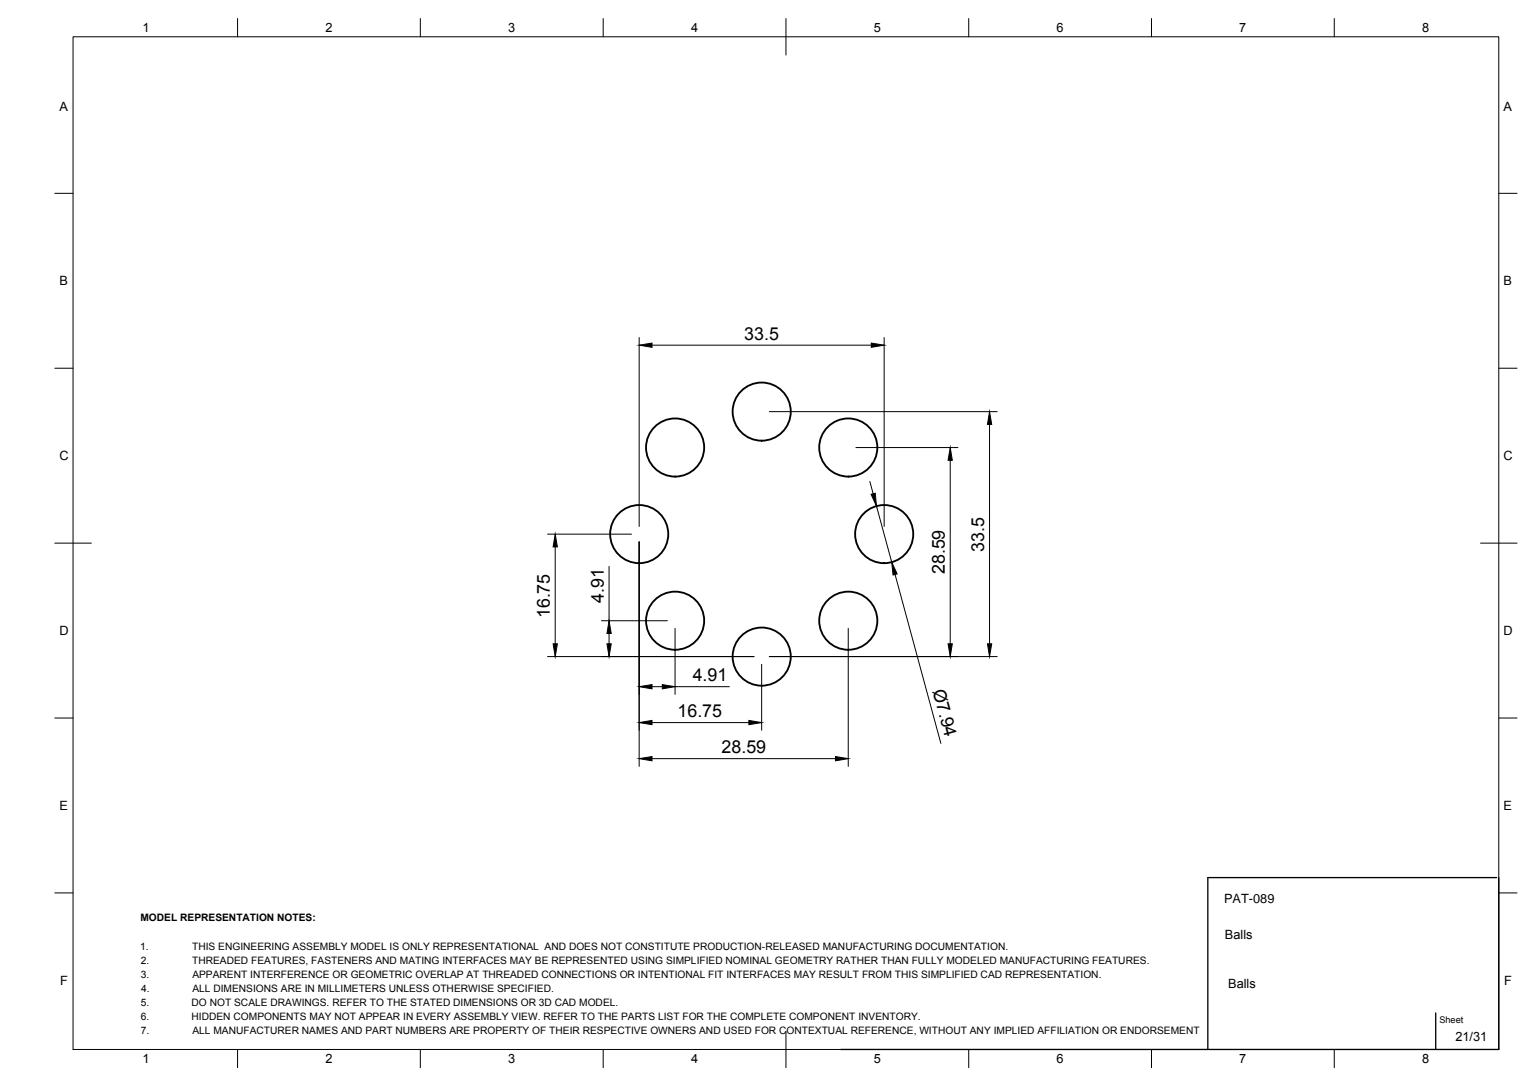
ISO-10303-21;
HEADER;
/* Generated by software containing ST-Developer
 * from STEP Tools, Inc. (www.steptools.com) 
 */

FILE_DESCRIPTION(
/* description */ ('Rotary union on bearing shaft'),
/* implementation_level */ '2;1');

FILE_NAME(
/* name */ 'Balls.step',
/* time_stamp */ '2026-10-28T03:24:01-07:00',
/* author */ (''),
/* organization */ (''),
/* preprocessor_version */ 'ST-DEVELOPER v20.2',
/* originating_system */ 'Autodesk Translation Framework v15.17.0.0',
/* authorisation */ '');

FILE_SCHEMA (('AUTOMOTIVE_DESIGN { 1 0 10303 214 3 1 1 }'));
ENDSEC;

DATA;
#10=MECHANICAL_DESIGN_GEOMETRIC_PRESENTATION_REPRESENTATION('',(#326,#327,#328,#329,#330,#331,#332,#333),#9448);
#185=SPHERICAL_SURFACE('',#5469,0.3969);
#186=SPHERICAL_SURFACE('',#5471,0.3969);
#187=SPHERICAL_SURFACE('',#5473,0.3969);
#188=SPHERICAL_SURFACE('',#5475,0.3969);
#189=SPHERICAL_SURFACE('',#5477,0.3969);
#190=SPHERICAL_SURFACE('',#5479,0.3969);
#191=SPHERICAL_SURFACE('',#5481,0.3969);
#192=SPHERICAL_SURFACE('',#5483,0.3969);
#272=SHAPE_REPRESENTATION_RELATIONSHIP('SRR','None',#9573,#299);
#299=ADVANCED_BREP_SHAPE_REPRESENTATION('',(#361,#362,#363,#364,#365,#366,
#367,#368),#9433);
#326=STYLED_ITEM('',(#9778),#361);
#327=STYLED_ITEM('',(#9778),#362);
#328=STYLED_ITEM('',(#9778),#363);
#329=STYLED_ITEM('',(#9778),#364);
#330=STYLED_ITEM('',(#9778),#365);
#331=STYLED_ITEM('',(#9778),#366);
#332=STYLED_ITEM('',(#9778),#367);
#333=STYLED_ITEM('',(#9778),#368);
#361=MANIFOLD_SOLID_BREP('Body1',#4881);
#362=MANIFOLD_SOLID_BREP('Body2',#4882);
#363=MANIFOLD_SOLID_BREP('Body3',#4883);
#364=MANIFOLD_SOLID_BREP('Body4',#4884);
#365=MANIFOLD_SOLID_BREP('Body5',#4885);
#366=MANIFOLD_SOLID_BREP('Body6',#4886);
#367=MANIFOLD_SOLID_BREP('Body7',#4887);
#368=MANIFOLD_SOLID_BREP('Body8',#4888);
#783=FACE_OUTER_BOUND('',#1150,.T.);
#784=FACE_OUTER_BOUND('',#1151,.T.);
#785=FACE_OUTER_BOUND('',#1152,.T.);
#786=FACE_OUTER_BOUND('',#1153,.T.);
#787=FACE_OUTER_BOUND('',#1154,.T.);
#788=FACE_OUTER_BOUND('',#1155,.T.);
#789=FACE_OUTER_BOUND('',#1156,.T.);
#790=FACE_OUTER_BOUND('',#1157,.T.);
#1150=EDGE_LOOP('',(#3787,#3788));
#1151=EDGE_LOOP('',(#3789,#3790));
#1152=EDGE_LOOP('',(#3791,#3792));
#1153=EDGE_LOOP('',(#3793,#3794));
#1154=EDGE_LOOP('',(#3795,#3796));
#1155=EDGE_LOOP('',(#3797,#3798));
#1156=EDGE_LOOP('',(#3799,#3800));
#1157=EDGE_LOOP('',(#3801,#3802));
#2122=CIRCLE('',#5470,0.3969);
#2123=CIRCLE('',#5472,0.3969);
#2124=CIRCLE('',#5474,0.3969);
#2125=CIRCLE('',#5476,0.3969);
#2126=CIRCLE('',#5478,0.3969);
#2127=CIRCLE('',#5480,0.3969);
#2128=CIRCLE('',#5482,0.3969);
#2129=CIRCLE('',#5484,0.3969);
#2424=VERTEX_POINT('',#8101);
#2425=VERTEX_POINT('',#8102);
#2426=VERTEX_POINT('',#8105);
#2427=VERTEX_POINT('',#8106);
#2428=VERTEX_POINT('',#8109);
#2429=VERTEX_POINT('',#8110);
#2430=VERTEX_POINT('',#8113);
#2431=VERTEX_POINT('',#8114);
#2432=VERTEX_POINT('',#8117);
#2433=VERTEX_POINT('',#8118);
#2434=VERTEX_POINT('',#8121);
#2435=VERTEX_POINT('',#8122);
#2436=VERTEX_POINT('',#8125);
#2437=VERTEX_POINT('',#8126);
#2438=VERTEX_POINT('',#8129);
#2439=VERTEX_POINT('',#8130);
#2921=EDGE_CURVE('',#2424,#2425,#2122,.T.);
#2922=EDGE_CURVE('',#2426,#2427,#2123,.T.);
#2923=EDGE_CURVE('',#2428,#2429,#2124,.T.);
#2924=EDGE_CURVE('',#2430,#2431,#2125,.T.);
#2925=EDGE_CURVE('',#2432,#2433,#2126,.T.);
#2926=EDGE_CURVE('',#2434,#2435,#2127,.T.);
#2927=EDGE_CURVE('',#2436,#2437,#2128,.T.);
#2928=EDGE_CURVE('',#2438,#2439,#2129,.T.);
#3787=ORIENTED_EDGE('',*,*,#2921,.T.);
#3788=ORIENTED_EDGE('',*,*,#2921,.F.);
#3789=ORIENTED_EDGE('',*,*,#2922,.T.);
#3790=ORIENTED_EDGE('',*,*,#2922,.F.);
#3791=ORIENTED_EDGE('',*,*,#2923,.T.);
#3792=ORIENTED_EDGE('',*,*,#2923,.F.);
#3793=ORIENTED_EDGE('',*,*,#2924,.T.);
#3794=ORIENTED_EDGE('',*,*,#2924,.F.);
#3795=ORIENTED_EDGE('',*,*,#2925,.T.);
#3796=ORIENTED_EDGE('',*,*,#2925,.F.);
#3797=ORIENTED_EDGE('',*,*,#2926,.T.);
#3798=ORIENTED_EDGE('',*,*,#2926,.F.);
#3799=ORIENTED_EDGE('',*,*,#2927,.T.);
#3800=ORIENTED_EDGE('',*,*,#2927,.F.);
#3801=ORIENTED_EDGE('',*,*,#2928,.T.);
#3802=ORIENTED_EDGE('',*,*,#2928,.F.);
#4696=ADVANCED_FACE('',(#783),#185,.T.);
#4697=ADVANCED_FACE('',(#784),#186,.T.);
#4698=ADVANCED_FACE('',(#785),#187,.T.);
#4699=ADVANCED_FACE('',(#786),#188,.T.);
#4700=ADVANCED_FACE('',(#787),#189,.T.);
#4701=ADVANCED_FACE('',(#788),#190,.T.);
#4702=ADVANCED_FACE('',(#789),#191,.T.);
#4703=ADVANCED_FACE('',(#790),#192,.T.);
#4881=CLOSED_SHELL('',(#4696));
#4882=CLOSED_SHELL('',(#4697));
#4883=CLOSED_SHELL('',(#4698));
#4884=CLOSED_SHELL('',(#4699));
#4885=CLOSED_SHELL('',(#4700));
#4886=CLOSED_SHELL('',(#4701));
#4887=CLOSED_SHELL('',(#4702));
#4888=CLOSED_SHELL('',(#4703));
#5468=AXIS2_PLACEMENT_3D('',#8099,#6487,#6488);
#5469=AXIS2_PLACEMENT_3D('',#8100,#6489,#6490);
#5470=AXIS2_PLACEMENT_3D('',#8103,#6491,#6492);
#5471=AXIS2_PLACEMENT_3D('',#8104,#6493,#6494);
#5472=AXIS2_PLACEMENT_3D('',#8107,#6495,#6496);
#5473=AXIS2_PLACEMENT_3D('',#8108,#6497,#6498);
#5474=AXIS2_PLACEMENT_3D('',#8111,#6499,#6500);
#5475=AXIS2_PLACEMENT_3D('',#8112,#6501,#6502);
#5476=AXIS2_PLACEMENT_3D('',#8115,#6503,#6504);
#5477=AXIS2_PLACEMENT_3D('',#8116,#6505,#6506);
#5478=AXIS2_PLACEMENT_3D('',#8119,#6507,#6508);
#5479=AXIS2_PLACEMENT_3D('',#8120,#6509,#6510);
#5480=AXIS2_PLACEMENT_3D('',#8123,#6511,#6512);
#5481=AXIS2_PLACEMENT_3D('',#8124,#6513,#6514);
#5482=AXIS2_PLACEMENT_3D('',#8127,#6515,#6516);
#5483=AXIS2_PLACEMENT_3D('',#8128,#6517,#6518);
#5484=AXIS2_PLACEMENT_3D('',#8131,#6519,#6520);
#6487=DIRECTION('axis',(0.,0.,1.));
#6488=DIRECTION('refdir',(1.,0.,0.));
#6489=DIRECTION('center_axis',(0.,0.,1.));
#6490=DIRECTION('ref_axis',(1.,0.,0.));
#6491=DIRECTION('center_axis',(1.22464679914735E-16,-1.,0.));
#6492=DIRECTION('ref_axis',(-1.,-1.22464679914735E-16,0.));
#6493=DIRECTION('center_axis',(0.707106781186548,0.,0.707106781186548));
#6494=DIRECTION('ref_axis',(0.707106781186548,0.,-0.707106781186548));
#6495=DIRECTION('center_axis',(8.65956056235493E-17,-1.,-8.65956056235493E-17));
#6496=DIRECTION('ref_axis',(-0.707106781186548,-1.22464679914735E-16,0.707106781186548));
#6497=DIRECTION('center_axis',(1.,0.,0.));
#6498=DIRECTION('ref_axis',(6.12323399573677E-17,0.,-1.));
#6499=DIRECTION('center_axis',(7.49879891330929E-33,-1.,-1.22464679914735E-16));
#6500=DIRECTION('ref_axis',(-6.12323399573677E-17,-1.22464679914735E-16,
1.));
#6501=DIRECTION('center_axis',(0.707106781186548,0.,-0.707106781186548));
#6502=DIRECTION('ref_axis',(-0.707106781186548,0.,-0.707106781186548));
#6503=DIRECTION('center_axis',(-8.65956056235493E-17,-1.,-8.65956056235493E-17));
#6504=DIRECTION('ref_axis',(0.707106781186548,-1.22464679914735E-16,0.707106781186548));
#6505=DIRECTION('center_axis',(0.,0.,-1.));
#6506=DIRECTION('ref_axis',(-1.,0.,-1.22464679914735E-16));
#6507=DIRECTION('center_axis',(-1.22464679914735E-16,-1.,-1.49975978266186E-32));
#6508=DIRECTION('ref_axis',(1.,-1.22464679914735E-16,1.22464679914735E-16));
#6509=DIRECTION('center_axis',(-0.707106781186548,0.,-0.707106781186548));
#6510=DIRECTION('ref_axis',(-0.707106781186548,0.,0.707106781186548));
#6511=DIRECTION('center_axis',(-8.65956056235493E-17,-1.,8.65956056235493E-17));
#6512=DIRECTION('ref_axis',(0.707106781186548,-1.22464679914735E-16,-0.707106781186548));
#6513=DIRECTION('center_axis',(-1.,0.,0.));
#6514=DIRECTION('ref_axis',(-1.83697019872103E-16,0.,1.));
#6515=DIRECTION('center_axis',(-2.24963967399279E-32,-1.,1.22464679914735E-16));
#6516=DIRECTION('ref_axis',(1.83697019872103E-16,-1.22464679914735E-16,
-1.));
#6517=DIRECTION('center_axis',(-0.707106781186548,0.,0.707106781186548));
#6518=DIRECTION('ref_axis',(0.707106781186548,0.,0.707106781186548));
#6519=DIRECTION('center_axis',(8.65956056235493E-17,-1.,8.65956056235494E-17));
#6520=DIRECTION('ref_axis',(-0.707106781186548,-1.22464679914735E-16,-0.707106781186548));
#8099=CARTESIAN_POINT('',(0.,0.,0.));
#8100=CARTESIAN_POINT('Origin',(1.675,0.,0.));
#8101=CARTESIAN_POINT('',(1.675,-2.97627328869245E-33,0.3969));
#8102=CARTESIAN_POINT('',(1.675,-2.97627328869245E-33,-0.3969));
#8103=CARTESIAN_POINT('Origin',(1.675,0.,0.));
#8104=CARTESIAN_POINT('Origin',(1.18440385848747,0.,-1.18440385848747));
#8105=CARTESIAN_POINT('',(1.46505453994041,3.1867025333467E-33,-0.903753177034526));
#8106=CARTESIAN_POINT('',(0.903753177034527,-9.13924911073161E-33,-1.46505453994041));
#8107=CARTESIAN_POINT('Origin',(1.18440385848747,0.,-1.18440385848747));
#8108=CARTESIAN_POINT('Origin',(1.02564169428591E-16,0.,-1.675));
#8109=CARTESIAN_POINT('',(0.3969,-2.97627328869246E-33,-1.675));
#8110=CARTESIAN_POINT('',(-0.3969,-2.97627328869245E-33,-1.675));
#8111=CARTESIAN_POINT('Origin',(1.02564169428591E-16,0.,-1.675));
#8112=CARTESIAN_POINT('Origin',(-1.18440385848747,0.,-1.18440385848747));
#8113=CARTESIAN_POINT('',(-0.903753177034526,3.1867025333467E-33,-1.46505453994041));
#8114=CARTESIAN_POINT('',(-1.46505453994041,-9.13924911073161E-33,-0.903753177034527));
#8115=CARTESIAN_POINT('Origin',(-1.18440385848747,0.,-1.18440385848747));
#8116=CARTESIAN_POINT('Origin',(-1.675,0.,-2.05128338857182E-16));
#8117=CARTESIAN_POINT('',(-1.675,-2.97627328869246E-33,-0.3969));
#8118=CARTESIAN_POINT('',(-1.675,-2.97627328869245E-33,0.3969));
#8119=CARTESIAN_POINT('Origin',(-1.675,0.,-2.05128338857182E-16));
#8120=CARTESIAN_POINT('Origin',(-1.18440385848747,0.,1.18440385848747));
#8121=CARTESIAN_POINT('',(-1.46505453994041,6.26819044436628E-33,0.903753177034526));
#8122=CARTESIAN_POINT('',(-0.903753177034527,-1.22207370217512E-32,1.46505453994041));
#8123=CARTESIAN_POINT('Origin',(-1.18440385848747,0.,1.18440385848747));
#8124=CARTESIAN_POINT('Origin',(-3.07692508285772E-16,0.,1.675));
#8125=CARTESIAN_POINT('',(-0.3969,-2.97627328869246E-33,1.675));
#8126=CARTESIAN_POINT('',(0.396899999999999,-2.97627328869245E-33,1.675));
#8127=CARTESIAN_POINT('Origin',(-3.07692508285772E-16,0.,1.675));
#8128=CARTESIAN_POINT('Origin',(1.18440385848747,0.,1.18440385848747));
#8129=CARTESIAN_POINT('',(0.903753177034526,9.34967835538585E-33,1.46505453994041));
#8130=CARTESIAN_POINT('',(1.46505453994041,-1.53022249327708E-32,0.903753177034527));
#8131=CARTESIAN_POINT('Origin',(1.18440385848747,0.,1.18440385848747));
#9401=UNCERTAINTY_MEASURE_WITH_UNIT(LENGTH_MEASURE(0.001),#9449,
'DISTANCE_ACCURACY_VALUE',
'Maximum model space distance between geometric entities at asserted c
onnectivities');
#9416=UNCERTAINTY_MEASURE_WITH_UNIT(LENGTH_MEASURE(0.001),#9449,
'DISTANCE_ACCURACY_VALUE',
'Maximum model space distance between geometric entities at asserted c
onnectivities');
#9433=(
GEOMETRIC_REPRESENTATION_CONTEXT(3)
GLOBAL_UNCERTAINTY_ASSIGNED_CONTEXT((#9401))
GLOBAL_UNIT_ASSIGNED_CONTEXT((#9449,#9451,#9452))
REPRESENTATION_CONTEXT('','3D')
);
#9448=(
GEOMETRIC_REPRESENTATION_CONTEXT(3)
GLOBAL_UNCERTAINTY_ASSIGNED_CONTEXT((#9416))
GLOBAL_UNIT_ASSIGNED_CONTEXT((#9449,#9451,#9452))
REPRESENTATION_CONTEXT('','3D')
);
#9449=(
LENGTH_UNIT()
NAMED_UNIT(*)
SI_UNIT(.CENTI.,.METRE.)
);
#9451=(
NAMED_UNIT(*)
PLANE_ANGLE_UNIT()
SI_UNIT($,.RADIAN.)
);
#9452=(
NAMED_UNIT(*)
SI_UNIT($,.STERADIAN.)
SOLID_ANGLE_UNIT()
);
#9469=SHAPE_DEFINITION_REPRESENTATION(#9500,#9573);
#9500=PRODUCT_DEFINITION_SHAPE('',$,#9605);
#9573=SHAPE_REPRESENTATION('',(#5468),#9433);
#9588=PRODUCT_DEFINITION_CONTEXT('part definition',#9683,'design');
#9605=PRODUCT_DEFINITION('Balls','Balls',#9636,#9588);
#9636=PRODUCT_DEFINITION_FORMATION('',$,#9701);
#9683=APPLICATION_CONTEXT(
'Core Data for Automotive Mechanical Design Process');
#9684=PRODUCT_CONTEXT('part definition',#9683,'mechanical');
#9701=PRODUCT('Balls','Balls','Balls',(#9684));
#9772=COLOUR_RGB('Grey',0.48,0.52,0.57);
#9773=FILL_AREA_STYLE_COLOUR('',#9772);
#9774=FILL_AREA_STYLE('',(#9773));
#9775=SURFACE_STYLE_FILL_AREA(#9774);
#9776=SURFACE_SIDE_STYLE('',(#9775));
#9777=SURFACE_STYLE_USAGE(.BOTH.,#9776);
#9778=PRESENTATION_STYLE_ASSIGNMENT((#9777));
ENDSEC;
END-ISO-10303-21;
